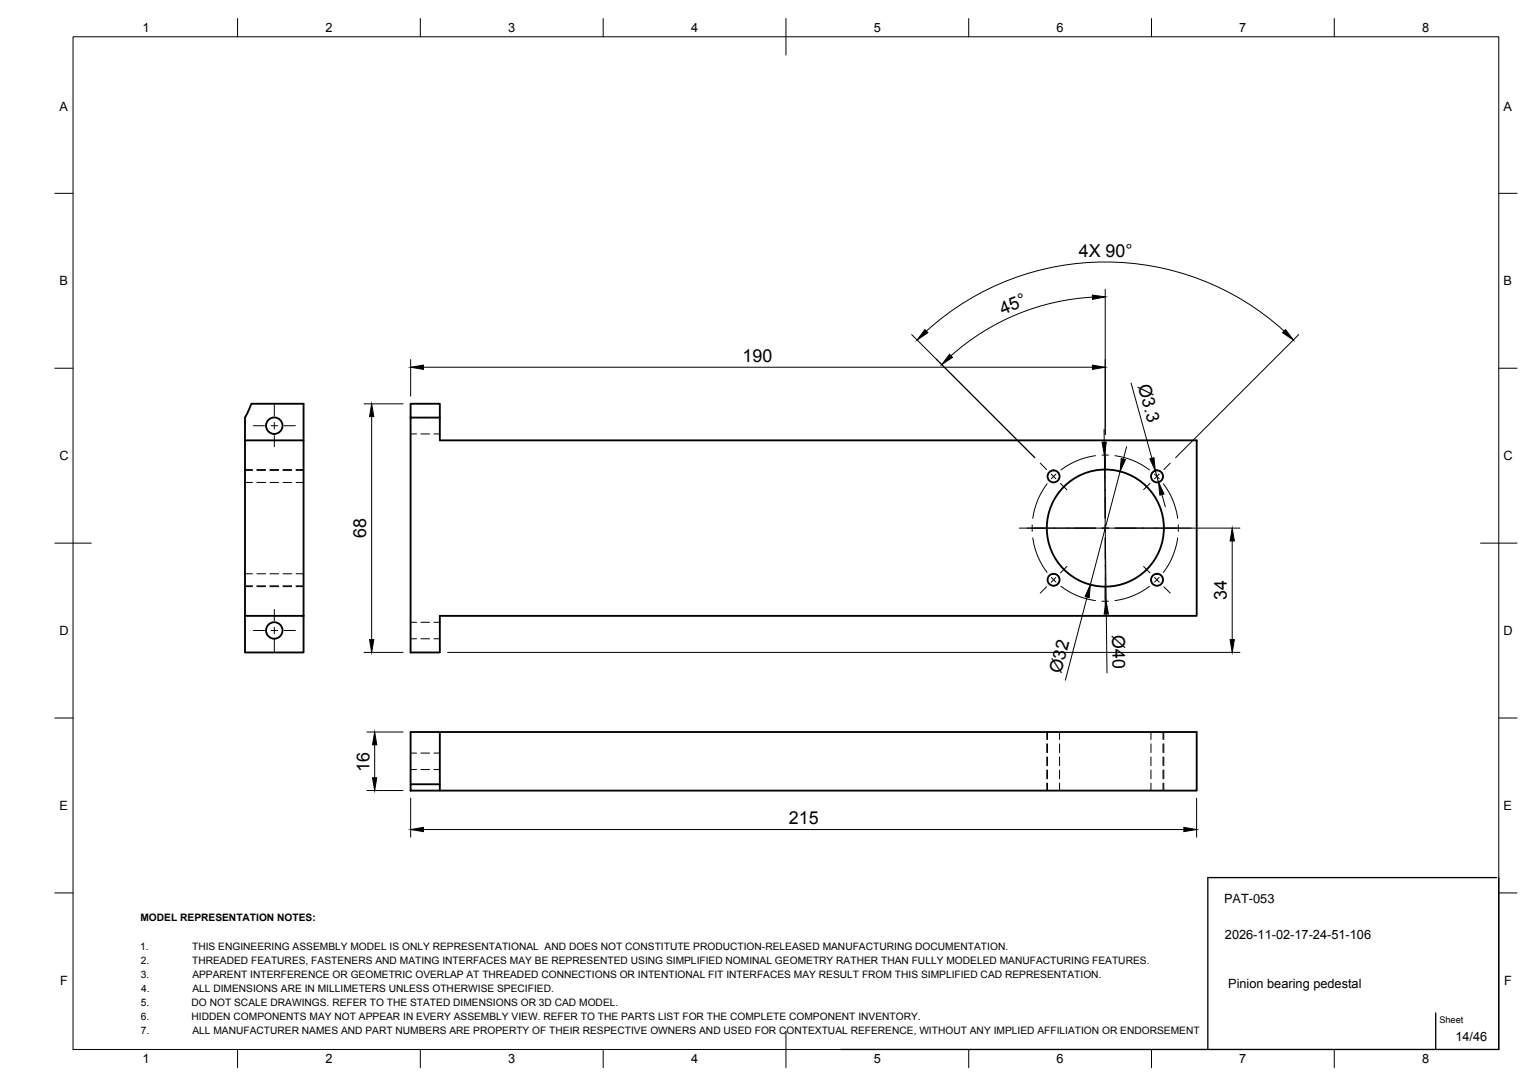
ISO-10303-21;
HEADER;
/* Generated by software containing ST-Developer
 * from STEP Tools, Inc. (www.steptools.com) 
 */

FILE_DESCRIPTION(
/* description */ ('Hand-operated arbor press'),
/* implementation_level */ '2;1');

FILE_NAME(
/* name */ 'Pinion bearing pedestal.step',
/* time_stamp */ '2026-10-28T03:25:25-07:00',
/* author */ (''),
/* organization */ (''),
/* preprocessor_version */ 'ST-DEVELOPER v20.2',
/* originating_system */ 'Autodesk Translation Framework v15.17.0.0',
/* authorisation */ '');

FILE_SCHEMA (('AUTOMOTIVE_DESIGN { 1 0 10303 214 3 1 1 }'));
ENDSEC;

DATA;
#10=MECHANICAL_DESIGN_GEOMETRIC_PRESENTATION_REPRESENTATION('',(#595),#32751);
#511=SHAPE_REPRESENTATION_RELATIONSHIP('SRR','None',#32940,#553);
#553=ADVANCED_BREP_SHAPE_REPRESENTATION('',(#644),#32714);
#595=STYLED_ITEM('',(#33242),#644);
#644=MANIFOLD_SOLID_BREP('Body1',#12492);
#729=FACE_BOUND('',#2151,.T.);
#730=FACE_BOUND('',#2152,.T.);
#731=FACE_BOUND('',#2162,.T.);
#732=FACE_BOUND('',#2164,.T.);
#733=FACE_BOUND('',#2167,.T.);
#734=FACE_BOUND('',#2168,.T.);
#735=FACE_BOUND('',#2169,.T.);
#736=FACE_BOUND('',#2170,.T.);
#737=FACE_BOUND('',#2171,.T.);
#738=FACE_BOUND('',#2174,.T.);
#739=FACE_BOUND('',#2175,.T.);
#740=FACE_BOUND('',#2176,.T.);
#741=FACE_BOUND('',#2177,.T.);
#742=FACE_BOUND('',#2178,.T.);
#934=PLANE('',#13222);
#935=PLANE('',#13225);
#936=PLANE('',#13245);
#937=PLANE('',#13246);
#938=PLANE('',#13247);
#939=PLANE('',#13248);
#940=PLANE('',#13249);
#941=PLANE('',#13250);
#942=PLANE('',#13251);
#943=PLANE('',#13252);
#1419=FACE_OUTER_BOUND('',#2149,.T.);
#1420=FACE_OUTER_BOUND('',#2150,.T.);
#1421=FACE_OUTER_BOUND('',#2153,.T.);
#1422=FACE_OUTER_BOUND('',#2154,.T.);
#1423=FACE_OUTER_BOUND('',#2155,.T.);
#1424=FACE_OUTER_BOUND('',#2156,.T.);
#1425=FACE_OUTER_BOUND('',#2157,.T.);
#1426=FACE_OUTER_BOUND('',#2158,.T.);
#1427=FACE_OUTER_BOUND('',#2159,.T.);
#1428=FACE_OUTER_BOUND('',#2160,.T.);
#1429=FACE_OUTER_BOUND('',#2161,.T.);
#1430=FACE_OUTER_BOUND('',#2163,.T.);
#1431=FACE_OUTER_BOUND('',#2165,.T.);
#1432=FACE_OUTER_BOUND('',#2166,.T.);
#1433=FACE_OUTER_BOUND('',#2172,.T.);
#1434=FACE_OUTER_BOUND('',#2173,.T.);
#1435=FACE_OUTER_BOUND('',#2179,.T.);
#1436=FACE_OUTER_BOUND('',#2180,.T.);
#2149=EDGE_LOOP('',(#8918,#8919,#8920,#8921));
#2150=EDGE_LOOP('',(#8922,#8923,#8924,#8925,#8926));
#2151=EDGE_LOOP('',(#8927));
#2152=EDGE_LOOP('',(#8928));
#2153=EDGE_LOOP('',(#8929,#8930,#8931,#8932));
#2154=EDGE_LOOP('',(#8933,#8934,#8935,#8936));
#2155=EDGE_LOOP('',(#8937,#8938,#8939,#8940));
#2156=EDGE_LOOP('',(#8941,#8942,#8943,#8944));
#2157=EDGE_LOOP('',(#8945,#8946,#8947,#8948));
#2158=EDGE_LOOP('',(#8949,#8950,#8951,#8952));
#2159=EDGE_LOOP('',(#8953,#8954,#8955,#8956));
#2160=EDGE_LOOP('',(#8957,#8958,#8959,#8960));
#2161=EDGE_LOOP('',(#8961,#8962,#8963,#8964,#8965));
#2162=EDGE_LOOP('',(#8966));
#2163=EDGE_LOOP('',(#8967,#8968,#8969,#8970));
#2164=EDGE_LOOP('',(#8971));
#2165=EDGE_LOOP('',(#8972,#8973,#8974,#8975));
#2166=EDGE_LOOP('',(#8976,#8977,#8978,#8979,#8980,#8981,#8982,#8983));
#2167=EDGE_LOOP('',(#8984));
#2168=EDGE_LOOP('',(#8985));
#2169=EDGE_LOOP('',(#8986));
#2170=EDGE_LOOP('',(#8987));
#2171=EDGE_LOOP('',(#8988));
#2172=EDGE_LOOP('',(#8989,#8990,#8991,#8992));
#2173=EDGE_LOOP('',(#8993,#8994,#8995,#8996,#8997,#8998,#8999,#9000));
#2174=EDGE_LOOP('',(#9001));
#2175=EDGE_LOOP('',(#9002));
#2176=EDGE_LOOP('',(#9003));
#2177=EDGE_LOOP('',(#9004));
#2178=EDGE_LOOP('',(#9005));
#2179=EDGE_LOOP('',(#9006,#9007,#9008,#9009));
#2180=EDGE_LOOP('',(#9010,#9011,#9012,#9013));
#3039=LINE('',#18276,#4210);
#3040=LINE('',#18279,#4211);
#3041=LINE('',#18282,#4212);
#3042=LINE('',#18284,#4213);
#3043=LINE('',#18286,#4214);
#3044=LINE('',#18287,#4215);
#3045=LINE('',#18294,#4216);
#3046=LINE('',#18295,#4217);
#3047=LINE('',#18300,#4218);
#3048=LINE('',#18306,#4219);
#3049=LINE('',#18312,#4220);
#3050=LINE('',#18318,#4221);
#3051=LINE('',#18322,#4222);
#3052=LINE('',#18326,#4223);
#3053=LINE('',#18332,#4224);
#3054=LINE('',#18336,#4225);
#3055=LINE('',#18338,#4226);
#3056=LINE('',#18339,#4227);
#3057=LINE('',#18343,#4228);
#3058=LINE('',#18345,#4229);
#3059=LINE('',#18347,#4230);
#3060=LINE('',#18348,#4231);
#3061=LINE('',#18350,#4232);
#3062=LINE('',#18351,#4233);
#3063=LINE('',#18354,#4234);
#3064=LINE('',#18356,#4235);
#3065=LINE('',#18357,#4236);
#3066=LINE('',#18360,#4237);
#3067=LINE('',#18361,#4238);
#3068=LINE('',#18364,#4239);
#3069=LINE('',#18365,#4240);
#3070=LINE('',#18367,#4241);
#4210=VECTOR('',#14814,1.);
#4211=VECTOR('',#14817,1.);
#4212=VECTOR('',#14820,1.);
#4213=VECTOR('',#14821,1.);
#4214=VECTOR('',#14822,1.);
#4215=VECTOR('',#14823,1.);
#4216=VECTOR('',#14830,1.);
#4217=VECTOR('',#14831,1.);
#4218=VECTOR('',#14836,0.165);
#4219=VECTOR('',#14843,0.165);
#4220=VECTOR('',#14850,0.165);
#4221=VECTOR('',#14857,0.165);
#4222=VECTOR('',#14862,0.225);
#4223=VECTOR('',#14867,0.225);
#4224=VECTOR('',#14874,1.6);
#4225=VECTOR('',#14879,1.);
#4226=VECTOR('',#14880,1.);
#4227=VECTOR('',#14881,1.);
#4228=VECTOR('',#14884,1.);
#4229=VECTOR('',#14885,1.);
#4230=VECTOR('',#14886,1.);
#4231=VECTOR('',#14887,1.);
#4232=VECTOR('',#14890,1.);
#4233=VECTOR('',#14891,1.);
#4234=VECTOR('',#14894,1.);
#4235=VECTOR('',#14895,1.);
#4236=VECTOR('',#14896,1.);
#4237=VECTOR('',#14899,1.);
#4238=VECTOR('',#14900,1.);
#4239=VECTOR('',#14903,1.);
#4240=VECTOR('',#14904,1.);
#4241=VECTOR('',#14907,1.);
#5248=CIRCLE('',#13220,2.52);
#5249=CIRCLE('',#13221,2.52);
#5250=CIRCLE('',#13223,0.225);
#5251=CIRCLE('',#13224,0.225);
#5252=CIRCLE('',#13227,0.165);
#5253=CIRCLE('',#13228,0.165);
#5254=CIRCLE('',#13230,0.165);
#5255=CIRCLE('',#13231,0.165);
#5256=CIRCLE('',#13233,0.165);
#5257=CIRCLE('',#13234,0.165);
#5258=CIRCLE('',#13236,0.165);
#5259=CIRCLE('',#13237,0.165);
#5260=CIRCLE('',#13239,0.225);
#5261=CIRCLE('',#13241,0.225);
#5262=CIRCLE('',#13243,1.6);
#5263=CIRCLE('',#13244,1.6);
#5754=VERTEX_POINT('',#18272);
#5755=VERTEX_POINT('',#18273);
#5756=VERTEX_POINT('',#18275);
#5757=VERTEX_POINT('',#18277);
#5758=VERTEX_POINT('',#18281);
#5759=VERTEX_POINT('',#18283);
#5760=VERTEX_POINT('',#18285);
#5761=VERTEX_POINT('',#18288);
#5762=VERTEX_POINT('',#18290);
#5763=VERTEX_POINT('',#18293);
#5764=VERTEX_POINT('',#18297);
#5765=VERTEX_POINT('',#18299);
#5766=VERTEX_POINT('',#18303);
#5767=VERTEX_POINT('',#18305);
#5768=VERTEX_POINT('',#18309);
#5769=VERTEX_POINT('',#18311);
#5770=VERTEX_POINT('',#18315);
#5771=VERTEX_POINT('',#18317);
#5772=VERTEX_POINT('',#18321);
#5773=VERTEX_POINT('',#18325);
#5774=VERTEX_POINT('',#18329);
#5775=VERTEX_POINT('',#18331);
#5776=VERTEX_POINT('',#18335);
#5777=VERTEX_POINT('',#18337);
#5778=VERTEX_POINT('',#18341);
#5779=VERTEX_POINT('',#18342);
#5780=VERTEX_POINT('',#18344);
#5781=VERTEX_POINT('',#18346);
#5782=VERTEX_POINT('',#18353);
#5783=VERTEX_POINT('',#18355);
#5784=VERTEX_POINT('',#18359);
#5785=VERTEX_POINT('',#18363);
#6962=EDGE_CURVE('',#5754,#5755,#5248,.T.);
#6963=EDGE_CURVE('',#5756,#5754,#3039,.T.);
#6964=EDGE_CURVE('',#5757,#5756,#5249,.T.);
#6965=EDGE_CURVE('',#5755,#5757,#3040,.T.);
#6966=EDGE_CURVE('',#5758,#5756,#3041,.T.);
#6967=EDGE_CURVE('',#5759,#5758,#3042,.T.);
#6968=EDGE_CURVE('',#5759,#5760,#3043,.T.);
#6969=EDGE_CURVE('',#5757,#5760,#3044,.T.);
#6970=EDGE_CURVE('',#5761,#5761,#5250,.T.);
#6971=EDGE_CURVE('',#5762,#5762,#5251,.T.);
#6972=EDGE_CURVE('',#5763,#5754,#3045,.T.);
#6973=EDGE_CURVE('',#5758,#5763,#3046,.T.);
#6974=EDGE_CURVE('',#5764,#5764,#5252,.T.);
#6975=EDGE_CURVE('',#5764,#5765,#3047,.T.);
#6976=EDGE_CURVE('',#5765,#5765,#5253,.T.);
#6977=EDGE_CURVE('',#5766,#5766,#5254,.T.);
#6978=EDGE_CURVE('',#5766,#5767,#3048,.T.);
#6979=EDGE_CURVE('',#5767,#5767,#5255,.T.);
#6980=EDGE_CURVE('',#5768,#5768,#5256,.T.);
#6981=EDGE_CURVE('',#5768,#5769,#3049,.T.);
#6982=EDGE_CURVE('',#5769,#5769,#5257,.T.);
#6983=EDGE_CURVE('',#5770,#5770,#5258,.T.);
#6984=EDGE_CURVE('',#5770,#5771,#3050,.T.);
#6985=EDGE_CURVE('',#5771,#5771,#5259,.T.);
#6986=EDGE_CURVE('',#5762,#5772,#3051,.T.);
#6987=EDGE_CURVE('',#5772,#5772,#5260,.T.);
#6988=EDGE_CURVE('',#5761,#5773,#3052,.T.);
#6989=EDGE_CURVE('',#5773,#5773,#5261,.T.);
#6990=EDGE_CURVE('',#5774,#5774,#5262,.T.);
#6991=EDGE_CURVE('',#5774,#5775,#3053,.T.);
#6992=EDGE_CURVE('',#5775,#5775,#5263,.T.);
#6993=EDGE_CURVE('',#5776,#5755,#3054,.T.);
#6994=EDGE_CURVE('',#5777,#5776,#3055,.T.);
#6995=EDGE_CURVE('',#5763,#5777,#3056,.T.);
#6996=EDGE_CURVE('',#5778,#5779,#3057,.T.);
#6997=EDGE_CURVE('',#5780,#5778,#3058,.T.);
#6998=EDGE_CURVE('',#5781,#5780,#3059,.T.);
#6999=EDGE_CURVE('',#5779,#5781,#3060,.T.);
#7000=EDGE_CURVE('',#5781,#5759,#3061,.T.);
#7001=EDGE_CURVE('',#5760,#5780,#3062,.T.);
#7002=EDGE_CURVE('',#5777,#5782,#3063,.T.);
#7003=EDGE_CURVE('',#5783,#5782,#3064,.T.);
#7004=EDGE_CURVE('',#5779,#5783,#3065,.T.);
#7005=EDGE_CURVE('',#5776,#5784,#3066,.T.);
#7006=EDGE_CURVE('',#5782,#5784,#3067,.T.);
#7007=EDGE_CURVE('',#5778,#5785,#3068,.T.);
#7008=EDGE_CURVE('',#5784,#5785,#3069,.T.);
#7009=EDGE_CURVE('',#5785,#5783,#3070,.T.);
#8918=ORIENTED_EDGE('',*,*,#6962,.F.);
#8919=ORIENTED_EDGE('',*,*,#6963,.F.);
#8920=ORIENTED_EDGE('',*,*,#6964,.F.);
#8921=ORIENTED_EDGE('',*,*,#6965,.F.);
#8922=ORIENTED_EDGE('',*,*,#6964,.T.);
#8923=ORIENTED_EDGE('',*,*,#6966,.F.);
#8924=ORIENTED_EDGE('',*,*,#6967,.F.);
#8925=ORIENTED_EDGE('',*,*,#6968,.T.);
#8926=ORIENTED_EDGE('',*,*,#6969,.F.);
#8927=ORIENTED_EDGE('',*,*,#6970,.T.);
#8928=ORIENTED_EDGE('',*,*,#6971,.T.);
#8929=ORIENTED_EDGE('',*,*,#6963,.T.);
#8930=ORIENTED_EDGE('',*,*,#6972,.F.);
#8931=ORIENTED_EDGE('',*,*,#6973,.F.);
#8932=ORIENTED_EDGE('',*,*,#6966,.T.);
#8933=ORIENTED_EDGE('',*,*,#6974,.F.);
#8934=ORIENTED_EDGE('',*,*,#6975,.T.);
#8935=ORIENTED_EDGE('',*,*,#6976,.F.);
#8936=ORIENTED_EDGE('',*,*,#6975,.F.);
#8937=ORIENTED_EDGE('',*,*,#6977,.F.);
#8938=ORIENTED_EDGE('',*,*,#6978,.T.);
#8939=ORIENTED_EDGE('',*,*,#6979,.F.);
#8940=ORIENTED_EDGE('',*,*,#6978,.F.);
#8941=ORIENTED_EDGE('',*,*,#6980,.F.);
#8942=ORIENTED_EDGE('',*,*,#6981,.T.);
#8943=ORIENTED_EDGE('',*,*,#6982,.F.);
#8944=ORIENTED_EDGE('',*,*,#6981,.F.);
#8945=ORIENTED_EDGE('',*,*,#6983,.F.);
#8946=ORIENTED_EDGE('',*,*,#6984,.T.);
#8947=ORIENTED_EDGE('',*,*,#6985,.F.);
#8948=ORIENTED_EDGE('',*,*,#6984,.F.);
#8949=ORIENTED_EDGE('',*,*,#6971,.F.);
#8950=ORIENTED_EDGE('',*,*,#6986,.T.);
#8951=ORIENTED_EDGE('',*,*,#6987,.F.);
#8952=ORIENTED_EDGE('',*,*,#6986,.F.);
#8953=ORIENTED_EDGE('',*,*,#6970,.F.);
#8954=ORIENTED_EDGE('',*,*,#6988,.T.);
#8955=ORIENTED_EDGE('',*,*,#6989,.F.);
#8956=ORIENTED_EDGE('',*,*,#6988,.F.);
#8957=ORIENTED_EDGE('',*,*,#6990,.F.);
#8958=ORIENTED_EDGE('',*,*,#6991,.T.);
#8959=ORIENTED_EDGE('',*,*,#6992,.F.);
#8960=ORIENTED_EDGE('',*,*,#6991,.F.);
#8961=ORIENTED_EDGE('',*,*,#6962,.T.);
#8962=ORIENTED_EDGE('',*,*,#6993,.F.);
#8963=ORIENTED_EDGE('',*,*,#6994,.F.);
#8964=ORIENTED_EDGE('',*,*,#6995,.F.);
#8965=ORIENTED_EDGE('',*,*,#6972,.T.);
#8966=ORIENTED_EDGE('',*,*,#6989,.T.);
#8967=ORIENTED_EDGE('',*,*,#6996,.F.);
#8968=ORIENTED_EDGE('',*,*,#6997,.F.);
#8969=ORIENTED_EDGE('',*,*,#6998,.F.);
#8970=ORIENTED_EDGE('',*,*,#6999,.F.);
#8971=ORIENTED_EDGE('',*,*,#6987,.T.);
#8972=ORIENTED_EDGE('',*,*,#7000,.F.);
#8973=ORIENTED_EDGE('',*,*,#6998,.T.);
#8974=ORIENTED_EDGE('',*,*,#7001,.F.);
#8975=ORIENTED_EDGE('',*,*,#6968,.F.);
#8976=ORIENTED_EDGE('',*,*,#7002,.T.);
#8977=ORIENTED_EDGE('',*,*,#7003,.F.);
#8978=ORIENTED_EDGE('',*,*,#7004,.F.);
#8979=ORIENTED_EDGE('',*,*,#6999,.T.);
#8980=ORIENTED_EDGE('',*,*,#7000,.T.);
#8981=ORIENTED_EDGE('',*,*,#6967,.T.);
#8982=ORIENTED_EDGE('',*,*,#6973,.T.);
#8983=ORIENTED_EDGE('',*,*,#6995,.T.);
#8984=ORIENTED_EDGE('',*,*,#6990,.T.);
#8985=ORIENTED_EDGE('',*,*,#6983,.T.);
#8986=ORIENTED_EDGE('',*,*,#6980,.T.);
#8987=ORIENTED_EDGE('',*,*,#6977,.T.);
#8988=ORIENTED_EDGE('',*,*,#6974,.T.);
#8989=ORIENTED_EDGE('',*,*,#6994,.T.);
#8990=ORIENTED_EDGE('',*,*,#7005,.T.);
#8991=ORIENTED_EDGE('',*,*,#7006,.F.);
#8992=ORIENTED_EDGE('',*,*,#7002,.F.);
#8993=ORIENTED_EDGE('',*,*,#6965,.T.);
#8994=ORIENTED_EDGE('',*,*,#6969,.T.);
#8995=ORIENTED_EDGE('',*,*,#7001,.T.);
#8996=ORIENTED_EDGE('',*,*,#6997,.T.);
#8997=ORIENTED_EDGE('',*,*,#7007,.T.);
#8998=ORIENTED_EDGE('',*,*,#7008,.F.);
#8999=ORIENTED_EDGE('',*,*,#7005,.F.);
#9000=ORIENTED_EDGE('',*,*,#6993,.T.);
#9001=ORIENTED_EDGE('',*,*,#6992,.T.);
#9002=ORIENTED_EDGE('',*,*,#6985,.T.);
#9003=ORIENTED_EDGE('',*,*,#6982,.T.);
#9004=ORIENTED_EDGE('',*,*,#6979,.T.);
#9005=ORIENTED_EDGE('',*,*,#6976,.T.);
#9006=ORIENTED_EDGE('',*,*,#6996,.T.);
#9007=ORIENTED_EDGE('',*,*,#7004,.T.);
#9008=ORIENTED_EDGE('',*,*,#7009,.F.);
#9009=ORIENTED_EDGE('',*,*,#7007,.F.);
#9010=ORIENTED_EDGE('',*,*,#7009,.T.);
#9011=ORIENTED_EDGE('',*,*,#7003,.T.);
#9012=ORIENTED_EDGE('',*,*,#7006,.T.);
#9013=ORIENTED_EDGE('',*,*,#7008,.T.);
#11683=CYLINDRICAL_SURFACE('',#13219,2.52);
#11684=CYLINDRICAL_SURFACE('',#13226,0.165);
#11685=CYLINDRICAL_SURFACE('',#13229,0.165);
#11686=CYLINDRICAL_SURFACE('',#13232,0.165);
#11687=CYLINDRICAL_SURFACE('',#13235,0.165);
#11688=CYLINDRICAL_SURFACE('',#13238,0.225);
#11689=CYLINDRICAL_SURFACE('',#13240,0.225);
#11690=CYLINDRICAL_SURFACE('',#13242,1.6);
#11928=ADVANCED_FACE('',(#1419),#11683,.F.);
#11929=ADVANCED_FACE('',(#1420,#729,#730),#934,.F.);
#11930=ADVANCED_FACE('',(#1421),#935,.T.);
#11931=ADVANCED_FACE('',(#1422),#11684,.F.);
#11932=ADVANCED_FACE('',(#1423),#11685,.F.);
#11933=ADVANCED_FACE('',(#1424),#11686,.F.);
#11934=ADVANCED_FACE('',(#1425),#11687,.F.);
#11935=ADVANCED_FACE('',(#1426),#11688,.F.);
#11936=ADVANCED_FACE('',(#1427),#11689,.F.);
#11937=ADVANCED_FACE('',(#1428),#11690,.F.);
#11938=ADVANCED_FACE('',(#1429,#731),#936,.T.);
#11939=ADVANCED_FACE('',(#1430,#732),#937,.T.);
#11940=ADVANCED_FACE('',(#1431),#938,.T.);
#11941=ADVANCED_FACE('',(#1432,#733,#734,#735,#736,#737),#939,.T.);
#11942=ADVANCED_FACE('',(#1433),#940,.T.);
#11943=ADVANCED_FACE('',(#1434,#738,#739,#740,#741,#742),#941,.T.);
#11944=ADVANCED_FACE('',(#1435),#942,.T.);
#11945=ADVANCED_FACE('',(#1436),#943,.T.);
#12492=CLOSED_SHELL('',(#11928,#11929,#11930,#11931,#11932,#11933,#11934,
#11935,#11936,#11937,#11938,#11939,#11940,#11941,#11942,#11943,#11944,#11945));
#13218=AXIS2_PLACEMENT_3D('',#18270,#14808,#14809);
#13219=AXIS2_PLACEMENT_3D('',#18271,#14810,#14811);
#13220=AXIS2_PLACEMENT_3D('',#18274,#14812,#14813);
#13221=AXIS2_PLACEMENT_3D('',#18278,#14815,#14816);
#13222=AXIS2_PLACEMENT_3D('',#18280,#14818,#14819);
#13223=AXIS2_PLACEMENT_3D('',#18289,#14824,#14825);
#13224=AXIS2_PLACEMENT_3D('',#18291,#14826,#14827);
#13225=AXIS2_PLACEMENT_3D('',#18292,#14828,#14829);
#13226=AXIS2_PLACEMENT_3D('',#18296,#14832,#14833);
#13227=AXIS2_PLACEMENT_3D('',#18298,#14834,#14835);
#13228=AXIS2_PLACEMENT_3D('',#18301,#14837,#14838);
#13229=AXIS2_PLACEMENT_3D('',#18302,#14839,#14840);
#13230=AXIS2_PLACEMENT_3D('',#18304,#14841,#14842);
#13231=AXIS2_PLACEMENT_3D('',#18307,#14844,#14845);
#13232=AXIS2_PLACEMENT_3D('',#18308,#14846,#14847);
#13233=AXIS2_PLACEMENT_3D('',#18310,#14848,#14849);
#13234=AXIS2_PLACEMENT_3D('',#18313,#14851,#14852);
#13235=AXIS2_PLACEMENT_3D('',#18314,#14853,#14854);
#13236=AXIS2_PLACEMENT_3D('',#18316,#14855,#14856);
#13237=AXIS2_PLACEMENT_3D('',#18319,#14858,#14859);
#13238=AXIS2_PLACEMENT_3D('',#18320,#14860,#14861);
#13239=AXIS2_PLACEMENT_3D('',#18323,#14863,#14864);
#13240=AXIS2_PLACEMENT_3D('',#18324,#14865,#14866);
#13241=AXIS2_PLACEMENT_3D('',#18327,#14868,#14869);
#13242=AXIS2_PLACEMENT_3D('',#18328,#14870,#14871);
#13243=AXIS2_PLACEMENT_3D('',#18330,#14872,#14873);
#13244=AXIS2_PLACEMENT_3D('',#18333,#14875,#14876);
#13245=AXIS2_PLACEMENT_3D('',#18334,#14877,#14878);
#13246=AXIS2_PLACEMENT_3D('',#18340,#14882,#14883);
#13247=AXIS2_PLACEMENT_3D('',#18349,#14888,#14889);
#13248=AXIS2_PLACEMENT_3D('',#18352,#14892,#14893);
#13249=AXIS2_PLACEMENT_3D('',#18358,#14897,#14898);
#13250=AXIS2_PLACEMENT_3D('',#18362,#14901,#14902);
#13251=AXIS2_PLACEMENT_3D('',#18366,#14905,#14906);
#13252=AXIS2_PLACEMENT_3D('',#18368,#14908,#14909);
#14808=DIRECTION('axis',(0.,0.,1.));
#14809=DIRECTION('refdir',(1.,0.,0.));
#14810=DIRECTION('center_axis',(0.,0.,1.));
#14811=DIRECTION('ref_axis',(1.,0.,0.));
#14812=DIRECTION('center_axis',(0.,0.,-1.));
#14813=DIRECTION('ref_axis',(1.,0.,0.));
#14814=DIRECTION('',(0.,0.,1.));
#14815=DIRECTION('center_axis',(0.,0.,1.));
#14816=DIRECTION('ref_axis',(1.,0.,0.));
#14817=DIRECTION('',(0.,0.,-1.));
#14818=DIRECTION('center_axis',(0.,0.,1.));
#14819=DIRECTION('ref_axis',(1.,0.,0.));
#14820=DIRECTION('',(0.,1.,0.));
#14821=DIRECTION('',(1.,0.,0.));
#14822=DIRECTION('',(0.,1.,0.));
#14823=DIRECTION('',(-1.,0.,0.));
#14824=DIRECTION('center_axis',(0.,0.,1.));
#14825=DIRECTION('ref_axis',(1.,0.,0.));
#14826=DIRECTION('center_axis',(0.,0.,1.));
#14827=DIRECTION('ref_axis',(1.,0.,0.));
#14828=DIRECTION('center_axis',(1.,0.,0.));
#14829=DIRECTION('ref_axis',(0.,0.,-1.));
#14830=DIRECTION('',(0.,1.,0.));
#14831=DIRECTION('',(0.,0.,1.));
#14832=DIRECTION('center_axis',(0.,1.,0.));
#14833=DIRECTION('ref_axis',(1.,0.,0.));
#14834=DIRECTION('center_axis',(0.,1.,0.));
#14835=DIRECTION('ref_axis',(1.,0.,0.));
#14836=DIRECTION('',(0.,1.,0.));
#14837=DIRECTION('center_axis',(0.,-1.,0.));
#14838=DIRECTION('ref_axis',(1.,0.,0.));
#14839=DIRECTION('center_axis',(0.,1.,0.));
#14840=DIRECTION('ref_axis',(1.,0.,0.));
#14841=DIRECTION('center_axis',(0.,1.,0.));
#14842=DIRECTION('ref_axis',(1.,0.,0.));
#14843=DIRECTION('',(0.,1.,0.));
#14844=DIRECTION('center_axis',(0.,-1.,0.));
#14845=DIRECTION('ref_axis',(1.,0.,0.));
#14846=DIRECTION('center_axis',(0.,1.,0.));
#14847=DIRECTION('ref_axis',(1.,0.,0.));
#14848=DIRECTION('center_axis',(0.,1.,0.));
#14849=DIRECTION('ref_axis',(1.,0.,0.));
#14850=DIRECTION('',(0.,1.,0.));
#14851=DIRECTION('center_axis',(0.,-1.,0.));
#14852=DIRECTION('ref_axis',(1.,0.,0.));
#14853=DIRECTION('center_axis',(0.,1.,0.));
#14854=DIRECTION('ref_axis',(1.,0.,0.));
#14855=DIRECTION('center_axis',(0.,1.,0.));
#14856=DIRECTION('ref_axis',(1.,0.,0.));
#14857=DIRECTION('',(0.,1.,0.));
#14858=DIRECTION('center_axis',(0.,-1.,0.));
#14859=DIRECTION('ref_axis',(1.,0.,0.));
#14860=DIRECTION('center_axis',(0.,0.,1.));
#14861=DIRECTION('ref_axis',(1.,0.,0.));
#14862=DIRECTION('',(0.,0.,1.));
#14863=DIRECTION('center_axis',(0.,0.,-1.));
#14864=DIRECTION('ref_axis',(1.,0.,0.));
#14865=DIRECTION('center_axis',(0.,0.,1.));
#14866=DIRECTION('ref_axis',(1.,0.,0.));
#14867=DIRECTION('',(0.,0.,1.));
#14868=DIRECTION('center_axis',(0.,0.,-1.));
#14869=DIRECTION('ref_axis',(1.,0.,0.));
#14870=DIRECTION('center_axis',(0.,1.,0.));
#14871=DIRECTION('ref_axis',(1.,0.,0.));
#14872=DIRECTION('center_axis',(0.,1.,0.));
#14873=DIRECTION('ref_axis',(1.,0.,0.));
#14874=DIRECTION('',(0.,1.,0.));
#14875=DIRECTION('center_axis',(0.,-1.,0.));
#14876=DIRECTION('ref_axis',(1.,0.,0.));
#14877=DIRECTION('center_axis',(0.,0.,1.));
#14878=DIRECTION('ref_axis',(1.,0.,0.));
#14879=DIRECTION('',(1.,0.,0.));
#14880=DIRECTION('',(0.,1.,0.));
#14881=DIRECTION('',(-1.,0.,0.));
#14882=DIRECTION('center_axis',(0.,0.,1.));
#14883=DIRECTION('ref_axis',(1.,0.,0.));
#14884=DIRECTION('',(0.,-1.,0.));
#14885=DIRECTION('',(1.,0.,0.));
#14886=DIRECTION('',(0.,1.,0.));
#14887=DIRECTION('',(-1.,0.,0.));
#14888=DIRECTION('center_axis',(-1.,0.,0.));
#14889=DIRECTION('ref_axis',(0.,0.,1.));
#14890=DIRECTION('',(0.,0.,-1.));
#14891=DIRECTION('',(0.,0.,1.));
#14892=DIRECTION('center_axis',(0.,-1.,0.));
#14893=DIRECTION('ref_axis',(1.,0.,0.));
#14894=DIRECTION('',(0.,0.,1.));
#14895=DIRECTION('',(1.,0.,0.));
#14896=DIRECTION('',(0.,0.,1.));
#14897=DIRECTION('center_axis',(1.,0.,0.));
#14898=DIRECTION('ref_axis',(0.,1.,0.));
#14899=DIRECTION('',(0.,0.,1.));
#14900=DIRECTION('',(0.,1.,0.));
#14901=DIRECTION('center_axis',(0.,1.,0.));
#14902=DIRECTION('ref_axis',(-1.,0.,0.));
#14903=DIRECTION('',(0.,0.,1.));
#14904=DIRECTION('',(-1.,0.,0.));
#14905=DIRECTION('center_axis',(-1.,0.,0.));
#14906=DIRECTION('ref_axis',(0.,-1.,0.));
#14907=DIRECTION('',(0.,-1.,0.));
#14908=DIRECTION('center_axis',(0.,0.,1.));
#14909=DIRECTION('ref_axis',(1.,0.,0.));
#18270=CARTESIAN_POINT('',(0.,0.,0.));
#18271=CARTESIAN_POINT('Origin',(1.,0.,0.9));
#18272=CARTESIAN_POINT('',(0.15,-2.37231954002828,1.8));
#18273=CARTESIAN_POINT('',(-0.228983319658977,-2.2,1.8));
#18274=CARTESIAN_POINT('Origin',(1.,0.,1.8));
#18275=CARTESIAN_POINT('',(0.15,-2.37231954002828,1.));
#18276=CARTESIAN_POINT('',(0.15,-2.37231954002828,0.9));
#18277=CARTESIAN_POINT('',(-0.228983319658977,-2.2,1.));
#18278=CARTESIAN_POINT('Origin',(1.,0.,1.));
#18279=CARTESIAN_POINT('',(-0.228983319658977,-2.2,0.9));
#18280=CARTESIAN_POINT('Origin',(-3.25,-3.,1.));
#18281=CARTESIAN_POINT('',(0.15,-3.8,1.));
#18282=CARTESIAN_POINT('',(0.15,-3.8,1.));
#18283=CARTESIAN_POINT('',(-6.65,-3.8,1.));
#18284=CARTESIAN_POINT('',(-6.65,-3.8,1.));
#18285=CARTESIAN_POINT('',(-6.65,-2.2,1.));
#18286=CARTESIAN_POINT('',(-6.65,-3.8,1.));
#18287=CARTESIAN_POINT('',(-6.65,-2.2,1.));
#18288=CARTESIAN_POINT('',(-0.675,-3.,1.));
#18289=CARTESIAN_POINT('Origin',(-0.45,-3.,1.));
#18290=CARTESIAN_POINT('',(-6.275,-3.,1.));
#18291=CARTESIAN_POINT('Origin',(-6.05,-3.,1.));
#18292=CARTESIAN_POINT('Origin',(0.15,-3.8,1.8));
#18293=CARTESIAN_POINT('',(0.15,-3.8,1.8));
#18294=CARTESIAN_POINT('',(0.15,-3.8,1.8));
#18295=CARTESIAN_POINT('',(0.15,-3.8,1.));
#18296=CARTESIAN_POINT('Origin',(-4.66421356237309,-3.9,18.5857864376269));
#18297=CARTESIAN_POINT('',(-4.82921356237309,-3.8,18.5857864376269));
#18298=CARTESIAN_POINT('Origin',(-4.66421356237309,-3.8,18.5857864376269));
#18299=CARTESIAN_POINT('',(-4.82921356237309,-2.2,18.5857864376269));
#18300=CARTESIAN_POINT('',(-4.82921356237309,-3.9,18.5857864376269));
#18301=CARTESIAN_POINT('Origin',(-4.66421356237309,-2.2,18.5857864376269));
#18302=CARTESIAN_POINT('Origin',(-4.66421356237309,-3.9,21.4142135623731));
#18303=CARTESIAN_POINT('',(-4.82921356237309,-3.8,21.4142135623731));
#18304=CARTESIAN_POINT('Origin',(-4.66421356237309,-3.8,21.4142135623731));
#18305=CARTESIAN_POINT('',(-4.82921356237309,-2.2,21.4142135623731));
#18306=CARTESIAN_POINT('',(-4.82921356237309,-3.9,21.4142135623731));
#18307=CARTESIAN_POINT('Origin',(-4.66421356237309,-2.2,21.4142135623731));
#18308=CARTESIAN_POINT('Origin',(-1.8357864376269,-3.9,21.4142135623731));
#18309=CARTESIAN_POINT('',(-2.00078643762691,-3.8,21.4142135623731));
#18310=CARTESIAN_POINT('Origin',(-1.8357864376269,-3.8,21.4142135623731));
#18311=CARTESIAN_POINT('',(-2.00078643762691,-2.2,21.4142135623731));
#18312=CARTESIAN_POINT('',(-2.00078643762691,-3.9,21.4142135623731));
#18313=CARTESIAN_POINT('Origin',(-1.8357864376269,-2.2,21.4142135623731));
#18314=CARTESIAN_POINT('Origin',(-1.83578643762691,-3.9,18.5857864376269));
#18315=CARTESIAN_POINT('',(-2.00078643762691,-3.8,18.5857864376269));
#18316=CARTESIAN_POINT('Origin',(-1.83578643762691,-3.8,18.5857864376269));
#18317=CARTESIAN_POINT('',(-2.00078643762691,-2.2,18.5857864376269));
#18318=CARTESIAN_POINT('',(-2.00078643762691,-3.9,18.5857864376269));
#18319=CARTESIAN_POINT('Origin',(-1.83578643762691,-2.2,18.5857864376269));
#18320=CARTESIAN_POINT('Origin',(-6.05,-3.,0.9));
#18321=CARTESIAN_POINT('',(-6.275,-3.,1.8));
#18322=CARTESIAN_POINT('',(-6.275,-3.,0.9));
#18323=CARTESIAN_POINT('Origin',(-6.05,-3.,1.8));
#18324=CARTESIAN_POINT('Origin',(-0.45,-3.,0.9));
#18325=CARTESIAN_POINT('',(-0.675,-3.,1.8));
#18326=CARTESIAN_POINT('',(-0.675,-3.,0.9));
#18327=CARTESIAN_POINT('Origin',(-0.45,-3.,1.8));
#18328=CARTESIAN_POINT('Origin',(-3.25,-3.9,20.));
#18329=CARTESIAN_POINT('',(-4.85,-3.8,20.));
#18330=CARTESIAN_POINT('Origin',(-3.25,-3.8,20.));
#18331=CARTESIAN_POINT('',(-4.85,-2.2,20.));
#18332=CARTESIAN_POINT('',(-4.85,-3.9,20.));
#18333=CARTESIAN_POINT('Origin',(-3.25,-2.2,20.));
#18334=CARTESIAN_POINT('Origin',(-6.65,-3.8,1.8));
#18335=CARTESIAN_POINT('',(-0.85,-2.2,1.8));
#18336=CARTESIAN_POINT('',(0.15,-2.2,1.8));
#18337=CARTESIAN_POINT('',(-0.85,-3.8,1.8));
#18338=CARTESIAN_POINT('',(-0.85,-3.8,1.8));
#18339=CARTESIAN_POINT('',(0.15,-3.8,1.8));
#18340=CARTESIAN_POINT('Origin',(-6.65,-3.8,1.8));
#18341=CARTESIAN_POINT('',(-5.65,-2.2,1.8));
#18342=CARTESIAN_POINT('',(-5.65,-3.8,1.8));
#18343=CARTESIAN_POINT('',(-5.65,-3.,1.8));
#18344=CARTESIAN_POINT('',(-6.65,-2.2,1.8));
#18345=CARTESIAN_POINT('',(0.15,-2.2,1.8));
#18346=CARTESIAN_POINT('',(-6.65,-3.8,1.8));
#18347=CARTESIAN_POINT('',(-6.65,-3.8,1.8));
#18348=CARTESIAN_POINT('',(0.15,-3.8,1.8));
#18349=CARTESIAN_POINT('Origin',(-6.65,-3.8,1.));
#18350=CARTESIAN_POINT('',(-6.65,-3.8,1.8));
#18351=CARTESIAN_POINT('',(-6.65,-2.2,1.8));
#18352=CARTESIAN_POINT('Origin',(-5.65,-3.8,1.));
#18353=CARTESIAN_POINT('',(-0.85,-3.8,22.5));
#18354=CARTESIAN_POINT('',(-0.85,-3.8,1.));
#18355=CARTESIAN_POINT('',(-5.65,-3.8,22.5));
#18356=CARTESIAN_POINT('',(-5.65,-3.8,22.5));
#18357=CARTESIAN_POINT('',(-5.65,-3.8,1.));
#18358=CARTESIAN_POINT('Origin',(-0.85,-3.8,1.));
#18359=CARTESIAN_POINT('',(-0.85,-2.2,22.5));
#18360=CARTESIAN_POINT('',(-0.85,-2.2,1.));
#18361=CARTESIAN_POINT('',(-0.85,-3.8,22.5));
#18362=CARTESIAN_POINT('Origin',(-0.85,-2.2,1.));
#18363=CARTESIAN_POINT('',(-5.65,-2.2,22.5));
#18364=CARTESIAN_POINT('',(-5.65,-2.2,1.));
#18365=CARTESIAN_POINT('',(-0.85,-2.2,22.5));
#18366=CARTESIAN_POINT('Origin',(-5.65,-2.2,1.));
#18367=CARTESIAN_POINT('',(-5.65,-2.2,22.5));
#18368=CARTESIAN_POINT('Origin',(-3.25,-3.,22.5));
#32665=UNCERTAINTY_MEASURE_WITH_UNIT(LENGTH_MEASURE(0.001),#32752,
'DISTANCE_ACCURACY_VALUE',
'Maximum model space distance between geometric entities at asserted c
onnectivities');
#32702=UNCERTAINTY_MEASURE_WITH_UNIT(LENGTH_MEASURE(0.001),#32752,
'DISTANCE_ACCURACY_VALUE',
'Maximum model space distance between geometric entities at asserted c
onnectivities');
#32714=(
GEOMETRIC_REPRESENTATION_CONTEXT(3)
GLOBAL_UNCERTAINTY_ASSIGNED_CONTEXT((#32665))
GLOBAL_UNIT_ASSIGNED_CONTEXT((#32752,#32754,#32755))
REPRESENTATION_CONTEXT('','3D')
);
#32751=(
GEOMETRIC_REPRESENTATION_CONTEXT(3)
GLOBAL_UNCERTAINTY_ASSIGNED_CONTEXT((#32702))
GLOBAL_UNIT_ASSIGNED_CONTEXT((#32752,#32754,#32755))
REPRESENTATION_CONTEXT('','3D')
);
#32752=(
LENGTH_UNIT()
NAMED_UNIT(*)
SI_UNIT(.CENTI.,.METRE.)
);
#32754=(
NAMED_UNIT(*)
PLANE_ANGLE_UNIT()
SI_UNIT($,.RADIAN.)
);
#32755=(
NAMED_UNIT(*)
SI_UNIT($,.STERADIAN.)
SOLID_ANGLE_UNIT()
);
#32767=SHAPE_DEFINITION_REPRESENTATION(#32815,#32940);
#32815=PRODUCT_DEFINITION_SHAPE('',$,#32989);
#32940=SHAPE_REPRESENTATION('',(#13218),#32714);
#32977=PRODUCT_DEFINITION_CONTEXT('part definition',#33123,'design');
#32989=PRODUCT_DEFINITION('Pinion bearing pedestal',
'Pinion bearing pedestal',#33037,#32977);
#33037=PRODUCT_DEFINITION_FORMATION('',$,#33136);
#33123=APPLICATION_CONTEXT(
'Core Data for Automotive Mechanical Design Process');
#33124=PRODUCT_CONTEXT('part definition',#33123,'mechanical');
#33136=PRODUCT('Pinion bearing pedestal','Pinion bearing pedestal',
'Pinion bearing pedestal',(#33124));
#33236=COLOUR_RGB('Grey',0.48,0.52,0.57);
#33237=FILL_AREA_STYLE_COLOUR('',#33236);
#33238=FILL_AREA_STYLE('',(#33237));
#33239=SURFACE_STYLE_FILL_AREA(#33238);
#33240=SURFACE_SIDE_STYLE('',(#33239));
#33241=SURFACE_STYLE_USAGE(.BOTH.,#33240);
#33242=PRESENTATION_STYLE_ASSIGNMENT((#33241));
ENDSEC;
END-ISO-10303-21;
